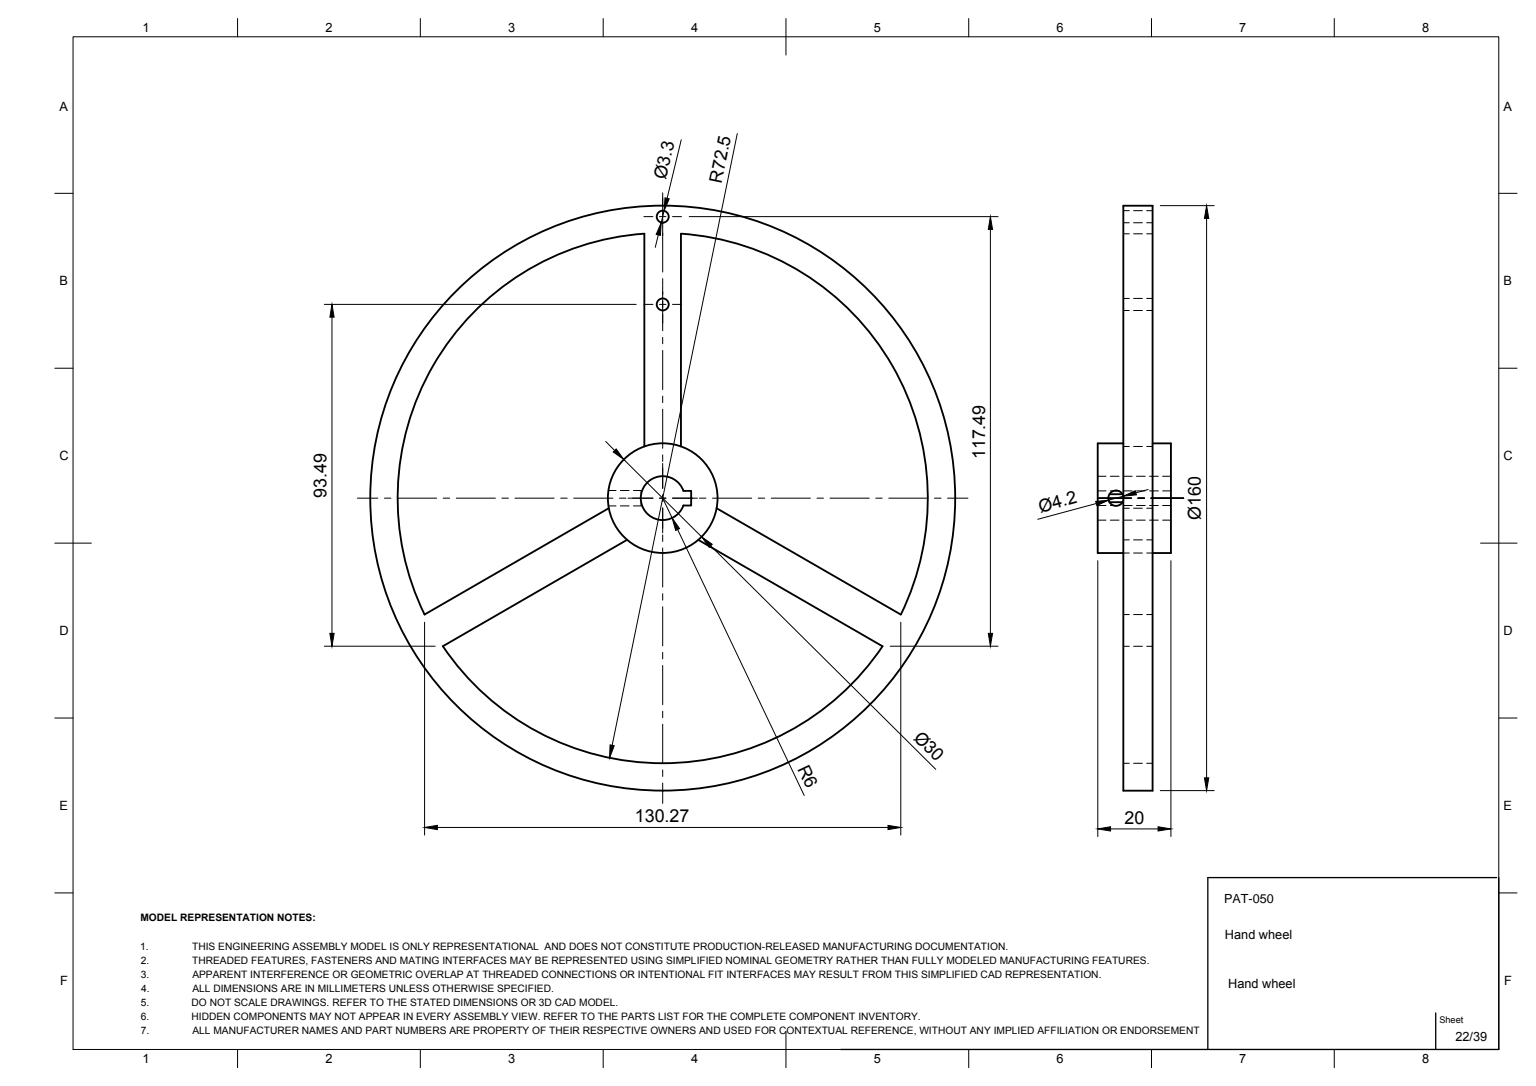
ISO-10303-21;
HEADER;
/* Generated by software containing ST-Developer
 * from STEP Tools, Inc. (www.steptools.com) 
 */

FILE_DESCRIPTION(
/* description */ ('Hand wheel with handle and shaft collar'),
/* implementation_level */ '2;1');

FILE_NAME(
/* name */ 'Hand wheel.step',
/* time_stamp */ '2026-10-28T03:23:19-07:00',
/* author */ (''),
/* organization */ (''),
/* preprocessor_version */ 'ST-DEVELOPER v20.2',
/* originating_system */ 'Autodesk Translation Framework v15.17.0.0',
/* authorisation */ '');

FILE_SCHEMA (('AUTOMOTIVE_DESIGN { 1 0 10303 214 3 1 1 }'));
ENDSEC;

DATA;
#10=MECHANICAL_DESIGN_GEOMETRIC_PRESENTATION_REPRESENTATION('',(#417),#10510);
#241=B_SPLINE_CURVE_WITH_KNOTS('',3,(#9168,#9169,#9170,#9171,#9172,#9173,
#9174,#9175,#9176,#9177),.UNSPECIFIED.,.F.,.F.,(4,2,2,2,4),(0.84783144568341,
0.878274576930948,0.958092875386314,1.03791117384168,1.06835430508922),
 .UNSPECIFIED.);
#242=B_SPLINE_CURVE_WITH_KNOTS('',3,(#9183,#9184,#9185,#9186,#9187,#9188,
#9189,#9190,#9191,#9192,#9193,#9194,#9195,#9196,#9197,#9198,#9199,#9200),
 .UNSPECIFIED.,.F.,.F.,(4,2,2,2,2,2,2,2,4),(0.,0.079216580773363,0.158433161546726,
0.23764869707457,0.316864232602414,0.396079768130259,0.475295303658103,
0.554511884431466,0.633728465204829),.UNSPECIFIED.);
#243=B_SPLINE_CURVE_WITH_KNOTS('',3,(#9201,#9202,#9203,#9204,#9205,#9206,
#9207,#9208,#9209,#9210,#9211,#9212,#9213,#9214,#9215,#9216,#9217,#9218),
 .UNSPECIFIED.,.F.,.F.,(4,2,2,2,2,2,2,2,4),(0.633728465204829,0.712945045978192,
0.792161626751555,0.871377162279399,0.950592697807243,1.02980823333509,
1.10902376886293,1.18824034963629,1.26745693040966),.UNSPECIFIED.);
#244=B_SPLINE_CURVE_WITH_KNOTS('',3,(#9221,#9222,#9223,#9224,#9225,#9226,
#9227,#9228,#9229,#9230),.UNSPECIFIED.,.F.,.F.,(4,2,2,2,4),(0.209102862092535,
0.239545993340072,0.319364291795438,0.399182590250804,0.429625721498342),
 .UNSPECIFIED.);
#346=SHAPE_REPRESENTATION_RELATIONSHIP('SRR','None',#10664,#378);
#378=ADVANCED_BREP_SHAPE_REPRESENTATION('',(#463),#10491);
#417=STYLED_ITEM('',(#10901),#463);
#463=MANIFOLD_SOLID_BREP('Body1',#5317);
#551=FACE_BOUND('',#1301,.T.);
#552=FACE_BOUND('',#1303,.T.);
#553=FACE_BOUND('',#1307,.T.);
#554=FACE_BOUND('',#1308,.T.);
#555=FACE_BOUND('',#1309,.T.);
#556=FACE_BOUND('',#1317,.T.);
#557=FACE_BOUND('',#1318,.T.);
#558=FACE_BOUND('',#1319,.T.);
#559=FACE_BOUND('',#1323,.T.);
#560=FACE_BOUND('',#1324,.T.);
#561=FACE_BOUND('',#1325,.T.);
#562=FACE_BOUND('',#1326,.T.);
#563=FACE_BOUND('',#1328,.T.);
#672=PLANE('',#6019);
#673=PLANE('',#6024);
#674=PLANE('',#6025);
#675=PLANE('',#6026);
#676=PLANE('',#6027);
#677=PLANE('',#6028);
#678=PLANE('',#6033);
#679=PLANE('',#6034);
#680=PLANE('',#6035);
#681=PLANE('',#6045);
#682=PLANE('',#6046);
#683=PLANE('',#6049);
#684=PLANE('',#6050);
#685=PLANE('',#6051);
#686=PLANE('',#6061);
#908=FACE_OUTER_BOUND('',#1292,.T.);
#909=FACE_OUTER_BOUND('',#1293,.T.);
#910=FACE_OUTER_BOUND('',#1294,.T.);
#911=FACE_OUTER_BOUND('',#1295,.T.);
#912=FACE_OUTER_BOUND('',#1296,.T.);
#913=FACE_OUTER_BOUND('',#1297,.T.);
#914=FACE_OUTER_BOUND('',#1298,.T.);
#915=FACE_OUTER_BOUND('',#1299,.T.);
#916=FACE_OUTER_BOUND('',#1300,.T.);
#917=FACE_OUTER_BOUND('',#1302,.T.);
#918=FACE_OUTER_BOUND('',#1304,.T.);
#919=FACE_OUTER_BOUND('',#1305,.T.);
#920=FACE_OUTER_BOUND('',#1306,.T.);
#921=FACE_OUTER_BOUND('',#1310,.T.);
#922=FACE_OUTER_BOUND('',#1311,.T.);
#923=FACE_OUTER_BOUND('',#1312,.T.);
#924=FACE_OUTER_BOUND('',#1313,.T.);
#925=FACE_OUTER_BOUND('',#1314,.T.);
#926=FACE_OUTER_BOUND('',#1315,.T.);
#927=FACE_OUTER_BOUND('',#1316,.T.);
#928=FACE_OUTER_BOUND('',#1320,.T.);
#929=FACE_OUTER_BOUND('',#1321,.T.);
#930=FACE_OUTER_BOUND('',#1322,.T.);
#931=FACE_OUTER_BOUND('',#1327,.T.);
#1292=EDGE_LOOP('',(#4163,#4164,#4165,#4166));
#1293=EDGE_LOOP('',(#4167,#4168,#4169,#4170));
#1294=EDGE_LOOP('',(#4171,#4172));
#1295=EDGE_LOOP('',(#4173,#4174,#4175,#4176,#4177,#4178,#4179,#4180,#4181));
#1296=EDGE_LOOP('',(#4182,#4183,#4184));
#1297=EDGE_LOOP('',(#4185,#4186,#4187,#4188));
#1298=EDGE_LOOP('',(#4189,#4190,#4191,#4192));
#1299=EDGE_LOOP('',(#4193,#4194,#4195,#4196));
#1300=EDGE_LOOP('',(#4197));
#1301=EDGE_LOOP('',(#4198,#4199,#4200,#4201));
#1302=EDGE_LOOP('',(#4202,#4203,#4204,#4205));
#1303=EDGE_LOOP('',(#4206,#4207,#4208,#4209));
#1304=EDGE_LOOP('',(#4210,#4211,#4212,#4213));
#1305=EDGE_LOOP('',(#4214,#4215,#4216,#4217));
#1306=EDGE_LOOP('',(#4218));
#1307=EDGE_LOOP('',(#4219));
#1308=EDGE_LOOP('',(#4220));
#1309=EDGE_LOOP('',(#4221,#4222,#4223,#4224,#4225,#4226,#4227,#4228,#4229,
#4230,#4231,#4232));
#1310=EDGE_LOOP('',(#4233,#4234,#4235,#4236));
#1311=EDGE_LOOP('',(#4237,#4238,#4239,#4240));
#1312=EDGE_LOOP('',(#4241,#4242,#4243,#4244));
#1313=EDGE_LOOP('',(#4245,#4246,#4247,#4248));
#1314=EDGE_LOOP('',(#4249,#4250,#4251,#4252));
#1315=EDGE_LOOP('',(#4253,#4254,#4255,#4256));
#1316=EDGE_LOOP('',(#4257));
#1317=EDGE_LOOP('',(#4258));
#1318=EDGE_LOOP('',(#4259));
#1319=EDGE_LOOP('',(#4260,#4261,#4262,#4263,#4264,#4265,#4266,#4267,#4268,
#4269,#4270,#4271));
#1320=EDGE_LOOP('',(#4272,#4273,#4274,#4275));
#1321=EDGE_LOOP('',(#4276,#4277,#4278,#4279));
#1322=EDGE_LOOP('',(#4280,#4281,#4282,#4283));
#1323=EDGE_LOOP('',(#4284,#4285));
#1324=EDGE_LOOP('',(#4286,#4287,#4288,#4289));
#1325=EDGE_LOOP('',(#4290,#4291,#4292,#4293));
#1326=EDGE_LOOP('',(#4294,#4295,#4296,#4297));
#1327=EDGE_LOOP('',(#4298));
#1328=EDGE_LOOP('',(#4299,#4300,#4301,#4302));
#1656=LINE('',#9153,#1966);
#1657=LINE('',#9159,#1967);
#1658=LINE('',#9164,#1968);
#1659=LINE('',#9181,#1969);
#1660=LINE('',#9232,#1970);
#1661=LINE('',#9236,#1971);
#1662=LINE('',#9238,#1972);
#1663=LINE('',#9240,#1973);
#1664=LINE('',#9241,#1974);
#1665=LINE('',#9244,#1975);
#1666=LINE('',#9246,#1976);
#1667=LINE('',#9247,#1977);
#1668=LINE('',#9250,#1978);
#1669=LINE('',#9252,#1979);
#1670=LINE('',#9253,#1980);
#1671=LINE('',#9263,#1981);
#1672=LINE('',#9265,#1982);
#1673=LINE('',#9267,#1983);
#1674=LINE('',#9268,#1984);
#1675=LINE('',#9272,#1985);
#1676=LINE('',#9274,#1986);
#1677=LINE('',#9276,#1987);
#1678=LINE('',#9277,#1988);
#1679=LINE('',#9284,#1989);
#1680=LINE('',#9288,#1990);
#1681=LINE('',#9292,#1991);
#1682=LINE('',#9296,#1992);
#1683=LINE('',#9302,#1993);
#1684=LINE('',#9305,#1994);
#1685=LINE('',#9306,#1995);
#1686=LINE('',#9309,#1996);
#1687=LINE('',#9311,#1997);
#1688=LINE('',#9312,#1998);
#1689=LINE('',#9316,#1999);
#1690=LINE('',#9319,#2000);
#1691=LINE('',#9320,#2001);
#1692=LINE('',#9323,#2002);
#1693=LINE('',#9325,#2003);
#1694=LINE('',#9326,#2004);
#1695=LINE('',#9336,#2005);
#1696=LINE('',#9339,#2006);
#1966=VECTOR('',#7198,0.165);
#1967=VECTOR('',#7205,0.165);
#1968=VECTOR('',#7210,1.);
#1969=VECTOR('',#7217,0.21);
#1970=VECTOR('',#7222,1.);
#1971=VECTOR('',#7225,1.);
#1972=VECTOR('',#7226,1.);
#1973=VECTOR('',#7227,1.);
#1974=VECTOR('',#7228,1.);
#1975=VECTOR('',#7231,1.);
#1976=VECTOR('',#7232,1.);
#1977=VECTOR('',#7233,1.);
#1978=VECTOR('',#7236,1.);
#1979=VECTOR('',#7237,1.);
#1980=VECTOR('',#7238,1.);
#1981=VECTOR('',#7251,1.);
#1982=VECTOR('',#7252,1.);
#1983=VECTOR('',#7253,1.);
#1984=VECTOR('',#7254,1.);
#1985=VECTOR('',#7257,1.);
#1986=VECTOR('',#7258,1.);
#1987=VECTOR('',#7259,1.);
#1988=VECTOR('',#7260,1.);
#1989=VECTOR('',#7267,1.);
#1990=VECTOR('',#7270,1.);
#1991=VECTOR('',#7273,1.);
#1992=VECTOR('',#7276,1.);
#1993=VECTOR('',#7285,1.);
#1994=VECTOR('',#7288,1.);
#1995=VECTOR('',#7289,1.);
#1996=VECTOR('',#7292,1.);
#1997=VECTOR('',#7293,1.);
#1998=VECTOR('',#7294,1.);
#1999=VECTOR('',#7299,1.);
#2000=VECTOR('',#7302,1.);
#2001=VECTOR('',#7303,1.);
#2002=VECTOR('',#7306,1.);
#2003=VECTOR('',#7307,1.);
#2004=VECTOR('',#7308,1.);
#2005=VECTOR('',#7325,8.);
#2006=VECTOR('',#7328,1.5);
#2279=CIRCLE('',#6014,0.165);
#2280=CIRCLE('',#6015,0.165);
#2281=CIRCLE('',#6017,0.165);
#2282=CIRCLE('',#6018,0.165);
#2283=CIRCLE('',#6020,0.21);
#2284=CIRCLE('',#6022,0.21);
#2285=CIRCLE('',#6023,0.21);
#2286=CIRCLE('',#6029,1.5);
#2287=CIRCLE('',#6030,0.6);
#2288=CIRCLE('',#6032,0.6);
#2289=CIRCLE('',#6036,8.);
#2290=CIRCLE('',#6037,7.25);
#2291=CIRCLE('',#6038,1.5);
#2292=CIRCLE('',#6039,7.25);
#2293=CIRCLE('',#6040,1.5);
#2294=CIRCLE('',#6041,7.25);
#2295=CIRCLE('',#6042,1.5);
#2296=CIRCLE('',#6044,7.25);
#2297=CIRCLE('',#6048,7.25);
#2298=CIRCLE('',#6052,8.);
#2299=CIRCLE('',#6053,7.25);
#2300=CIRCLE('',#6054,1.5);
#2301=CIRCLE('',#6055,1.5);
#2302=CIRCLE('',#6056,1.5);
#2303=CIRCLE('',#6060,1.5);
#2653=VERTEX_POINT('',#9150);
#2654=VERTEX_POINT('',#9152);
#2655=VERTEX_POINT('',#9156);
#2656=VERTEX_POINT('',#9158);
#2657=VERTEX_POINT('',#9162);
#2658=VERTEX_POINT('',#9163);
#2659=VERTEX_POINT('',#9167);
#2660=VERTEX_POINT('',#9178);
#2661=VERTEX_POINT('',#9180);
#2662=VERTEX_POINT('',#9182);
#2663=VERTEX_POINT('',#9219);
#2664=VERTEX_POINT('',#9234);
#2665=VERTEX_POINT('',#9235);
#2666=VERTEX_POINT('',#9237);
#2667=VERTEX_POINT('',#9239);
#2668=VERTEX_POINT('',#9243);
#2669=VERTEX_POINT('',#9245);
#2670=VERTEX_POINT('',#9249);
#2671=VERTEX_POINT('',#9251);
#2672=VERTEX_POINT('',#9255);
#2673=VERTEX_POINT('',#9261);
#2674=VERTEX_POINT('',#9262);
#2675=VERTEX_POINT('',#9264);
#2676=VERTEX_POINT('',#9266);
#2677=VERTEX_POINT('',#9270);
#2678=VERTEX_POINT('',#9271);
#2679=VERTEX_POINT('',#9273);
#2680=VERTEX_POINT('',#9275);
#2681=VERTEX_POINT('',#9279);
#2682=VERTEX_POINT('',#9281);
#2683=VERTEX_POINT('',#9283);
#2684=VERTEX_POINT('',#9285);
#2685=VERTEX_POINT('',#9287);
#2686=VERTEX_POINT('',#9289);
#2687=VERTEX_POINT('',#9291);
#2688=VERTEX_POINT('',#9293);
#2689=VERTEX_POINT('',#9295);
#2690=VERTEX_POINT('',#9300);
#2691=VERTEX_POINT('',#9304);
#2692=VERTEX_POINT('',#9308);
#2693=VERTEX_POINT('',#9310);
#2694=VERTEX_POINT('',#9314);
#2695=VERTEX_POINT('',#9318);
#2696=VERTEX_POINT('',#9322);
#2697=VERTEX_POINT('',#9324);
#2698=VERTEX_POINT('',#9328);
#2699=VERTEX_POINT('',#9338);
#3199=EDGE_CURVE('',#2653,#2653,#2279,.T.);
#3200=EDGE_CURVE('',#2653,#2654,#1656,.T.);
#3201=EDGE_CURVE('',#2654,#2654,#2280,.T.);
#3202=EDGE_CURVE('',#2655,#2655,#2281,.T.);
#3203=EDGE_CURVE('',#2655,#2656,#1657,.T.);
#3204=EDGE_CURVE('',#2656,#2656,#2282,.T.);
#3205=EDGE_CURVE('',#2657,#2658,#1658,.T.);
#3206=EDGE_CURVE('',#2657,#2658,#2283,.T.);
#3207=EDGE_CURVE('',#2659,#2657,#241,.T.);
#3208=EDGE_CURVE('',#2660,#2659,#2284,.T.);
#3209=EDGE_CURVE('',#2660,#2661,#1659,.T.);
#3210=EDGE_CURVE('',#2662,#2661,#242,.T.);
#3211=EDGE_CURVE('',#2661,#2662,#243,.T.);
#3212=EDGE_CURVE('',#2663,#2660,#2285,.T.);
#3213=EDGE_CURVE('',#2658,#2663,#244,.T.);
#3214=EDGE_CURVE('',#2663,#2659,#1660,.T.);
#3215=EDGE_CURVE('',#2664,#2665,#1661,.T.);
#3216=EDGE_CURVE('',#2664,#2666,#1662,.T.);
#3217=EDGE_CURVE('',#2667,#2666,#1663,.T.);
#3218=EDGE_CURVE('',#2665,#2667,#1664,.T.);
#3219=EDGE_CURVE('',#2668,#2664,#1665,.T.);
#3220=EDGE_CURVE('',#2668,#2669,#1666,.T.);
#3221=EDGE_CURVE('',#2666,#2669,#1667,.T.);
#3222=EDGE_CURVE('',#2670,#2668,#1668,.T.);
#3223=EDGE_CURVE('',#2671,#2670,#1669,.T.);
#3224=EDGE_CURVE('',#2669,#2671,#1670,.T.);
#3225=EDGE_CURVE('',#2672,#2672,#2286,.T.);
#3226=EDGE_CURVE('',#2671,#2667,#2287,.T.);
#3227=EDGE_CURVE('',#2670,#2665,#2288,.T.);
#3228=EDGE_CURVE('',#2673,#2674,#1671,.T.);
#3229=EDGE_CURVE('',#2675,#2673,#1672,.T.);
#3230=EDGE_CURVE('',#2676,#2675,#1673,.T.);
#3231=EDGE_CURVE('',#2674,#2676,#1674,.T.);
#3232=EDGE_CURVE('',#2677,#2678,#1675,.T.);
#3233=EDGE_CURVE('',#2679,#2677,#1676,.T.);
#3234=EDGE_CURVE('',#2680,#2679,#1677,.T.);
#3235=EDGE_CURVE('',#2678,#2680,#1678,.T.);
#3236=EDGE_CURVE('',#2681,#2681,#2289,.T.);
#3237=EDGE_CURVE('',#2682,#2677,#2290,.T.);
#3238=EDGE_CURVE('',#2682,#2683,#1679,.T.);
#3239=EDGE_CURVE('',#2684,#2683,#2291,.T.);
#3240=EDGE_CURVE('',#2684,#2685,#1680,.T.);
#3241=EDGE_CURVE('',#2686,#2685,#2292,.T.);
#3242=EDGE_CURVE('',#2686,#2687,#1681,.T.);
#3243=EDGE_CURVE('',#2688,#2687,#2293,.T.);
#3244=EDGE_CURVE('',#2688,#2689,#1682,.T.);
#3245=EDGE_CURVE('',#2674,#2689,#2294,.T.);
#3246=EDGE_CURVE('',#2679,#2676,#2295,.T.);
#3247=EDGE_CURVE('',#2690,#2678,#2296,.T.);
#3248=EDGE_CURVE('',#2690,#2682,#1683,.T.);
#3249=EDGE_CURVE('',#2691,#2690,#1684,.T.);
#3250=EDGE_CURVE('',#2683,#2691,#1685,.T.);
#3251=EDGE_CURVE('',#2685,#2692,#1686,.T.);
#3252=EDGE_CURVE('',#2693,#2684,#1687,.T.);
#3253=EDGE_CURVE('',#2692,#2693,#1688,.T.);
#3254=EDGE_CURVE('',#2694,#2692,#2297,.T.);
#3255=EDGE_CURVE('',#2694,#2686,#1689,.T.);
#3256=EDGE_CURVE('',#2687,#2695,#1690,.T.);
#3257=EDGE_CURVE('',#2695,#2694,#1691,.T.);
#3258=EDGE_CURVE('',#2696,#2688,#1692,.T.);
#3259=EDGE_CURVE('',#2697,#2696,#1693,.T.);
#3260=EDGE_CURVE('',#2689,#2697,#1694,.T.);
#3261=EDGE_CURVE('',#2698,#2698,#2298,.T.);
#3262=EDGE_CURVE('',#2673,#2697,#2299,.T.);
#3263=EDGE_CURVE('',#2695,#2696,#2300,.T.);
#3264=EDGE_CURVE('',#2691,#2693,#2301,.T.);
#3265=EDGE_CURVE('',#2675,#2680,#2302,.T.);
#3266=EDGE_CURVE('',#2698,#2681,#1695,.T.);
#3267=EDGE_CURVE('',#2672,#2699,#1696,.T.);
#3268=EDGE_CURVE('',#2699,#2699,#2303,.T.);
#4163=ORIENTED_EDGE('',*,*,#3199,.F.);
#4164=ORIENTED_EDGE('',*,*,#3200,.T.);
#4165=ORIENTED_EDGE('',*,*,#3201,.F.);
#4166=ORIENTED_EDGE('',*,*,#3200,.F.);
#4167=ORIENTED_EDGE('',*,*,#3202,.F.);
#4168=ORIENTED_EDGE('',*,*,#3203,.T.);
#4169=ORIENTED_EDGE('',*,*,#3204,.F.);
#4170=ORIENTED_EDGE('',*,*,#3203,.F.);
#4171=ORIENTED_EDGE('',*,*,#3205,.F.);
#4172=ORIENTED_EDGE('',*,*,#3206,.T.);
#4173=ORIENTED_EDGE('',*,*,#3207,.F.);
#4174=ORIENTED_EDGE('',*,*,#3208,.F.);
#4175=ORIENTED_EDGE('',*,*,#3209,.T.);
#4176=ORIENTED_EDGE('',*,*,#3210,.F.);
#4177=ORIENTED_EDGE('',*,*,#3211,.F.);
#4178=ORIENTED_EDGE('',*,*,#3209,.F.);
#4179=ORIENTED_EDGE('',*,*,#3212,.F.);
#4180=ORIENTED_EDGE('',*,*,#3213,.F.);
#4181=ORIENTED_EDGE('',*,*,#3206,.F.);
#4182=ORIENTED_EDGE('',*,*,#3214,.F.);
#4183=ORIENTED_EDGE('',*,*,#3212,.T.);
#4184=ORIENTED_EDGE('',*,*,#3208,.T.);
#4185=ORIENTED_EDGE('',*,*,#3215,.F.);
#4186=ORIENTED_EDGE('',*,*,#3216,.T.);
#4187=ORIENTED_EDGE('',*,*,#3217,.F.);
#4188=ORIENTED_EDGE('',*,*,#3218,.F.);
#4189=ORIENTED_EDGE('',*,*,#3219,.F.);
#4190=ORIENTED_EDGE('',*,*,#3220,.T.);
#4191=ORIENTED_EDGE('',*,*,#3221,.F.);
#4192=ORIENTED_EDGE('',*,*,#3216,.F.);
#4193=ORIENTED_EDGE('',*,*,#3222,.F.);
#4194=ORIENTED_EDGE('',*,*,#3223,.F.);
#4195=ORIENTED_EDGE('',*,*,#3224,.F.);
#4196=ORIENTED_EDGE('',*,*,#3220,.F.);
#4197=ORIENTED_EDGE('',*,*,#3225,.T.);
#4198=ORIENTED_EDGE('',*,*,#3217,.T.);
#4199=ORIENTED_EDGE('',*,*,#3221,.T.);
#4200=ORIENTED_EDGE('',*,*,#3224,.T.);
#4201=ORIENTED_EDGE('',*,*,#3226,.T.);
#4202=ORIENTED_EDGE('',*,*,#3218,.T.);
#4203=ORIENTED_EDGE('',*,*,#3226,.F.);
#4204=ORIENTED_EDGE('',*,*,#3223,.T.);
#4205=ORIENTED_EDGE('',*,*,#3227,.T.);
#4206=ORIENTED_EDGE('',*,*,#3213,.T.);
#4207=ORIENTED_EDGE('',*,*,#3214,.T.);
#4208=ORIENTED_EDGE('',*,*,#3207,.T.);
#4209=ORIENTED_EDGE('',*,*,#3205,.T.);
#4210=ORIENTED_EDGE('',*,*,#3228,.F.);
#4211=ORIENTED_EDGE('',*,*,#3229,.F.);
#4212=ORIENTED_EDGE('',*,*,#3230,.F.);
#4213=ORIENTED_EDGE('',*,*,#3231,.F.);
#4214=ORIENTED_EDGE('',*,*,#3232,.F.);
#4215=ORIENTED_EDGE('',*,*,#3233,.F.);
#4216=ORIENTED_EDGE('',*,*,#3234,.F.);
#4217=ORIENTED_EDGE('',*,*,#3235,.F.);
#4218=ORIENTED_EDGE('',*,*,#3236,.F.);
#4219=ORIENTED_EDGE('',*,*,#3199,.T.);
#4220=ORIENTED_EDGE('',*,*,#3202,.T.);
#4221=ORIENTED_EDGE('',*,*,#3237,.F.);
#4222=ORIENTED_EDGE('',*,*,#3238,.T.);
#4223=ORIENTED_EDGE('',*,*,#3239,.F.);
#4224=ORIENTED_EDGE('',*,*,#3240,.T.);
#4225=ORIENTED_EDGE('',*,*,#3241,.F.);
#4226=ORIENTED_EDGE('',*,*,#3242,.T.);
#4227=ORIENTED_EDGE('',*,*,#3243,.F.);
#4228=ORIENTED_EDGE('',*,*,#3244,.T.);
#4229=ORIENTED_EDGE('',*,*,#3245,.F.);
#4230=ORIENTED_EDGE('',*,*,#3231,.T.);
#4231=ORIENTED_EDGE('',*,*,#3246,.F.);
#4232=ORIENTED_EDGE('',*,*,#3233,.T.);
#4233=ORIENTED_EDGE('',*,*,#3232,.T.);
#4234=ORIENTED_EDGE('',*,*,#3247,.F.);
#4235=ORIENTED_EDGE('',*,*,#3248,.T.);
#4236=ORIENTED_EDGE('',*,*,#3237,.T.);
#4237=ORIENTED_EDGE('',*,*,#3248,.F.);
#4238=ORIENTED_EDGE('',*,*,#3249,.F.);
#4239=ORIENTED_EDGE('',*,*,#3250,.F.);
#4240=ORIENTED_EDGE('',*,*,#3238,.F.);
#4241=ORIENTED_EDGE('',*,*,#3251,.F.);
#4242=ORIENTED_EDGE('',*,*,#3240,.F.);
#4243=ORIENTED_EDGE('',*,*,#3252,.F.);
#4244=ORIENTED_EDGE('',*,*,#3253,.F.);
#4245=ORIENTED_EDGE('',*,*,#3251,.T.);
#4246=ORIENTED_EDGE('',*,*,#3254,.F.);
#4247=ORIENTED_EDGE('',*,*,#3255,.T.);
#4248=ORIENTED_EDGE('',*,*,#3241,.T.);
#4249=ORIENTED_EDGE('',*,*,#3256,.F.);
#4250=ORIENTED_EDGE('',*,*,#3242,.F.);
#4251=ORIENTED_EDGE('',*,*,#3255,.F.);
#4252=ORIENTED_EDGE('',*,*,#3257,.F.);
#4253=ORIENTED_EDGE('',*,*,#3258,.F.);
#4254=ORIENTED_EDGE('',*,*,#3259,.F.);
#4255=ORIENTED_EDGE('',*,*,#3260,.F.);
#4256=ORIENTED_EDGE('',*,*,#3244,.F.);
#4257=ORIENTED_EDGE('',*,*,#3261,.T.);
#4258=ORIENTED_EDGE('',*,*,#3201,.T.);
#4259=ORIENTED_EDGE('',*,*,#3204,.T.);
#4260=ORIENTED_EDGE('',*,*,#3262,.T.);
#4261=ORIENTED_EDGE('',*,*,#3259,.T.);
#4262=ORIENTED_EDGE('',*,*,#3263,.F.);
#4263=ORIENTED_EDGE('',*,*,#3257,.T.);
#4264=ORIENTED_EDGE('',*,*,#3254,.T.);
#4265=ORIENTED_EDGE('',*,*,#3253,.T.);
#4266=ORIENTED_EDGE('',*,*,#3264,.F.);
#4267=ORIENTED_EDGE('',*,*,#3249,.T.);
#4268=ORIENTED_EDGE('',*,*,#3247,.T.);
#4269=ORIENTED_EDGE('',*,*,#3235,.T.);
#4270=ORIENTED_EDGE('',*,*,#3265,.F.);
#4271=ORIENTED_EDGE('',*,*,#3229,.T.);
#4272=ORIENTED_EDGE('',*,*,#3228,.T.);
#4273=ORIENTED_EDGE('',*,*,#3245,.T.);
#4274=ORIENTED_EDGE('',*,*,#3260,.T.);
#4275=ORIENTED_EDGE('',*,*,#3262,.F.);
#4276=ORIENTED_EDGE('',*,*,#3261,.F.);
#4277=ORIENTED_EDGE('',*,*,#3266,.T.);
#4278=ORIENTED_EDGE('',*,*,#3236,.T.);
#4279=ORIENTED_EDGE('',*,*,#3266,.F.);
#4280=ORIENTED_EDGE('',*,*,#3225,.F.);
#4281=ORIENTED_EDGE('',*,*,#3267,.T.);
#4282=ORIENTED_EDGE('',*,*,#3268,.T.);
#4283=ORIENTED_EDGE('',*,*,#3267,.F.);
#4284=ORIENTED_EDGE('',*,*,#3210,.T.);
#4285=ORIENTED_EDGE('',*,*,#3211,.T.);
#4286=ORIENTED_EDGE('',*,*,#3230,.T.);
#4287=ORIENTED_EDGE('',*,*,#3265,.T.);
#4288=ORIENTED_EDGE('',*,*,#3234,.T.);
#4289=ORIENTED_EDGE('',*,*,#3246,.T.);
#4290=ORIENTED_EDGE('',*,*,#3250,.T.);
#4291=ORIENTED_EDGE('',*,*,#3264,.T.);
#4292=ORIENTED_EDGE('',*,*,#3252,.T.);
#4293=ORIENTED_EDGE('',*,*,#3239,.T.);
#4294=ORIENTED_EDGE('',*,*,#3256,.T.);
#4295=ORIENTED_EDGE('',*,*,#3263,.T.);
#4296=ORIENTED_EDGE('',*,*,#3258,.T.);
#4297=ORIENTED_EDGE('',*,*,#3243,.T.);
#4298=ORIENTED_EDGE('',*,*,#3268,.F.);
#4299=ORIENTED_EDGE('',*,*,#3215,.T.);
#4300=ORIENTED_EDGE('',*,*,#3227,.F.);
#4301=ORIENTED_EDGE('',*,*,#3222,.T.);
#4302=ORIENTED_EDGE('',*,*,#3219,.T.);
#4927=CYLINDRICAL_SURFACE('',#6013,0.165);
#4928=CYLINDRICAL_SURFACE('',#6016,0.165);
#4929=CYLINDRICAL_SURFACE('',#6021,0.21);
#4930=CYLINDRICAL_SURFACE('',#6031,0.6);
#4931=CYLINDRICAL_SURFACE('',#6043,7.25);
#4932=CYLINDRICAL_SURFACE('',#6047,7.25);
#4933=CYLINDRICAL_SURFACE('',#6057,7.25);
#4934=CYLINDRICAL_SURFACE('',#6058,8.);
#4935=CYLINDRICAL_SURFACE('',#6059,1.5);
#5120=ADVANCED_FACE('',(#908),#4927,.F.);
#5121=ADVANCED_FACE('',(#909),#4928,.F.);
#5122=ADVANCED_FACE('',(#910),#672,.T.);
#5123=ADVANCED_FACE('',(#911),#4929,.F.);
#5124=ADVANCED_FACE('',(#912),#673,.T.);
#5125=ADVANCED_FACE('',(#913),#674,.F.);
#5126=ADVANCED_FACE('',(#914),#675,.F.);
#5127=ADVANCED_FACE('',(#915),#676,.F.);
#5128=ADVANCED_FACE('',(#916,#551),#677,.T.);
#5129=ADVANCED_FACE('',(#917,#552),#4930,.F.);
#5130=ADVANCED_FACE('',(#918),#678,.T.);
#5131=ADVANCED_FACE('',(#919),#679,.T.);
#5132=ADVANCED_FACE('',(#920,#553,#554,#555),#680,.F.);
#5133=ADVANCED_FACE('',(#921),#4931,.F.);
#5134=ADVANCED_FACE('',(#922),#681,.T.);
#5135=ADVANCED_FACE('',(#923),#682,.T.);
#5136=ADVANCED_FACE('',(#924),#4932,.F.);
#5137=ADVANCED_FACE('',(#925),#683,.T.);
#5138=ADVANCED_FACE('',(#926),#684,.T.);
#5139=ADVANCED_FACE('',(#927,#556,#557,#558),#685,.T.);
#5140=ADVANCED_FACE('',(#928),#4933,.F.);
#5141=ADVANCED_FACE('',(#929),#4934,.T.);
#5142=ADVANCED_FACE('',(#930,#559,#560,#561,#562),#4935,.T.);
#5143=ADVANCED_FACE('',(#931,#563),#686,.F.);
#5317=CLOSED_SHELL('',(#5120,#5121,#5122,#5123,#5124,#5125,#5126,#5127,
#5128,#5129,#5130,#5131,#5132,#5133,#5134,#5135,#5136,#5137,#5138,#5139,
#5140,#5141,#5142,#5143));
#6012=AXIS2_PLACEMENT_3D('',#9148,#7192,#7193);
#6013=AXIS2_PLACEMENT_3D('',#9149,#7194,#7195);
#6014=AXIS2_PLACEMENT_3D('',#9151,#7196,#7197);
#6015=AXIS2_PLACEMENT_3D('',#9154,#7199,#7200);
#6016=AXIS2_PLACEMENT_3D('',#9155,#7201,#7202);
#6017=AXIS2_PLACEMENT_3D('',#9157,#7203,#7204);
#6018=AXIS2_PLACEMENT_3D('',#9160,#7206,#7207);
#6019=AXIS2_PLACEMENT_3D('',#9161,#7208,#7209);
#6020=AXIS2_PLACEMENT_3D('',#9165,#7211,#7212);
#6021=AXIS2_PLACEMENT_3D('',#9166,#7213,#7214);
#6022=AXIS2_PLACEMENT_3D('',#9179,#7215,#7216);
#6023=AXIS2_PLACEMENT_3D('',#9220,#7218,#7219);
#6024=AXIS2_PLACEMENT_3D('',#9231,#7220,#7221);
#6025=AXIS2_PLACEMENT_3D('',#9233,#7223,#7224);
#6026=AXIS2_PLACEMENT_3D('',#9242,#7229,#7230);
#6027=AXIS2_PLACEMENT_3D('',#9248,#7234,#7235);
#6028=AXIS2_PLACEMENT_3D('',#9254,#7239,#7240);
#6029=AXIS2_PLACEMENT_3D('',#9256,#7241,#7242);
#6030=AXIS2_PLACEMENT_3D('',#9257,#7243,#7244);
#6031=AXIS2_PLACEMENT_3D('',#9258,#7245,#7246);
#6032=AXIS2_PLACEMENT_3D('',#9259,#7247,#7248);
#6033=AXIS2_PLACEMENT_3D('',#9260,#7249,#7250);
#6034=AXIS2_PLACEMENT_3D('',#9269,#7255,#7256);
#6035=AXIS2_PLACEMENT_3D('',#9278,#7261,#7262);
#6036=AXIS2_PLACEMENT_3D('',#9280,#7263,#7264);
#6037=AXIS2_PLACEMENT_3D('',#9282,#7265,#7266);
#6038=AXIS2_PLACEMENT_3D('',#9286,#7268,#7269);
#6039=AXIS2_PLACEMENT_3D('',#9290,#7271,#7272);
#6040=AXIS2_PLACEMENT_3D('',#9294,#7274,#7275);
#6041=AXIS2_PLACEMENT_3D('',#9297,#7277,#7278);
#6042=AXIS2_PLACEMENT_3D('',#9298,#7279,#7280);
#6043=AXIS2_PLACEMENT_3D('',#9299,#7281,#7282);
#6044=AXIS2_PLACEMENT_3D('',#9301,#7283,#7284);
#6045=AXIS2_PLACEMENT_3D('',#9303,#7286,#7287);
#6046=AXIS2_PLACEMENT_3D('',#9307,#7290,#7291);
#6047=AXIS2_PLACEMENT_3D('',#9313,#7295,#7296);
#6048=AXIS2_PLACEMENT_3D('',#9315,#7297,#7298);
#6049=AXIS2_PLACEMENT_3D('',#9317,#7300,#7301);
#6050=AXIS2_PLACEMENT_3D('',#9321,#7304,#7305);
#6051=AXIS2_PLACEMENT_3D('',#9327,#7309,#7310);
#6052=AXIS2_PLACEMENT_3D('',#9329,#7311,#7312);
#6053=AXIS2_PLACEMENT_3D('',#9330,#7313,#7314);
#6054=AXIS2_PLACEMENT_3D('',#9331,#7315,#7316);
#6055=AXIS2_PLACEMENT_3D('',#9332,#7317,#7318);
#6056=AXIS2_PLACEMENT_3D('',#9333,#7319,#7320);
#6057=AXIS2_PLACEMENT_3D('',#9334,#7321,#7322);
#6058=AXIS2_PLACEMENT_3D('',#9335,#7323,#7324);
#6059=AXIS2_PLACEMENT_3D('',#9337,#7326,#7327);
#6060=AXIS2_PLACEMENT_3D('',#9340,#7329,#7330);
#6061=AXIS2_PLACEMENT_3D('',#9341,#7331,#7332);
#7192=DIRECTION('axis',(0.,0.,1.));
#7193=DIRECTION('refdir',(1.,0.,0.));
#7194=DIRECTION('center_axis',(0.,1.,0.));
#7195=DIRECTION('ref_axis',(1.,0.,0.));
#7196=DIRECTION('center_axis',(0.,1.,0.));
#7197=DIRECTION('ref_axis',(1.,0.,0.));
#7198=DIRECTION('',(0.,1.,0.));
#7199=DIRECTION('center_axis',(0.,-1.,0.));
#7200=DIRECTION('ref_axis',(1.,0.,0.));
#7201=DIRECTION('center_axis',(0.,1.,0.));
#7202=DIRECTION('ref_axis',(1.,0.,0.));
#7203=DIRECTION('center_axis',(0.,1.,0.));
#7204=DIRECTION('ref_axis',(1.,0.,0.));
#7205=DIRECTION('',(0.,1.,0.));
#7206=DIRECTION('center_axis',(0.,-1.,0.));
#7207=DIRECTION('ref_axis',(1.,0.,0.));
#7208=DIRECTION('center_axis',(0.,0.,1.));
#7209=DIRECTION('ref_axis',(1.,0.,0.));
#7210=DIRECTION('',(0.,1.,0.));
#7211=DIRECTION('center_axis',(0.,0.,1.));
#7212=DIRECTION('ref_axis',(1.,0.,0.));
#7213=DIRECTION('center_axis',(0.,0.,1.));
#7214=DIRECTION('ref_axis',(1.,0.,0.));
#7215=DIRECTION('center_axis',(0.,0.,1.));
#7216=DIRECTION('ref_axis',(1.,0.,0.));
#7217=DIRECTION('',(0.,0.,1.));
#7218=DIRECTION('center_axis',(0.,0.,1.));
#7219=DIRECTION('ref_axis',(1.,0.,0.));
#7220=DIRECTION('center_axis',(0.,0.,1.));
#7221=DIRECTION('ref_axis',(1.,0.,0.));
#7222=DIRECTION('',(0.,-1.,0.));
#7223=DIRECTION('center_axis',(-1.,0.,0.));
#7224=DIRECTION('ref_axis',(0.,0.,1.));
#7225=DIRECTION('',(0.,0.,1.));
#7226=DIRECTION('',(0.,1.,0.));
#7227=DIRECTION('',(0.,0.,-1.));
#7228=DIRECTION('',(0.,1.,0.));
#7229=DIRECTION('center_axis',(0.,0.,-1.));
#7230=DIRECTION('ref_axis',(-1.,0.,0.));
#7231=DIRECTION('',(-1.,0.,0.));
#7232=DIRECTION('',(0.,1.,0.));
#7233=DIRECTION('',(1.,0.,0.));
#7234=DIRECTION('center_axis',(1.,0.,0.));
#7235=DIRECTION('ref_axis',(0.,0.,-1.));
#7236=DIRECTION('',(0.,0.,-1.));
#7237=DIRECTION('',(0.,-1.,0.));
#7238=DIRECTION('',(0.,0.,1.));
#7239=DIRECTION('center_axis',(0.,1.,0.));
#7240=DIRECTION('ref_axis',(1.,0.,0.));
#7241=DIRECTION('center_axis',(0.,1.,0.));
#7242=DIRECTION('ref_axis',(1.,0.,0.));
#7243=DIRECTION('center_axis',(0.,-1.,0.));
#7244=DIRECTION('ref_axis',(1.,0.,0.));
#7245=DIRECTION('center_axis',(0.,1.,0.));
#7246=DIRECTION('ref_axis',(-1.83697019872103E-16,0.,1.));
#7247=DIRECTION('center_axis',(0.,-1.,0.));
#7248=DIRECTION('ref_axis',(1.,0.,0.));
#7249=DIRECTION('center_axis',(0.866025403784438,0.,-0.5));
#7250=DIRECTION('ref_axis',(-0.5,0.,-0.866025403784438));
#7251=DIRECTION('',(0.,-1.,0.));
#7252=DIRECTION('',(-0.5,0.,-0.866025403784438));
#7253=DIRECTION('',(0.,1.,0.));
#7254=DIRECTION('',(0.5,0.,0.866025403784438));
#7255=DIRECTION('center_axis',(-0.866025403784438,0.,0.5));
#7256=DIRECTION('ref_axis',(0.5,0.,0.866025403784438));
#7257=DIRECTION('',(0.,1.,0.));
#7258=DIRECTION('',(-0.5,0.,-0.866025403784438));
#7259=DIRECTION('',(0.,-1.,0.));
#7260=DIRECTION('',(0.5,0.,0.866025403784438));
#7261=DIRECTION('center_axis',(0.,1.,0.));
#7262=DIRECTION('ref_axis',(1.,0.,0.));
#7263=DIRECTION('center_axis',(0.,1.,0.));
#7264=DIRECTION('ref_axis',(1.,0.,0.));
#7265=DIRECTION('center_axis',(0.,-1.,0.));
#7266=DIRECTION('ref_axis',(1.,0.,0.));
#7267=DIRECTION('',(0.5,0.,-0.866025403784439));
#7268=DIRECTION('center_axis',(0.,-1.,0.));
#7269=DIRECTION('ref_axis',(1.,0.,0.));
#7270=DIRECTION('',(-0.5,0.,0.866025403784439));
#7271=DIRECTION('center_axis',(0.,-1.,0.));
#7272=DIRECTION('ref_axis',(1.,0.,0.));
#7273=DIRECTION('',(-1.,0.,0.));
#7274=DIRECTION('center_axis',(0.,-1.,0.));
#7275=DIRECTION('ref_axis',(1.,0.,0.));
#7276=DIRECTION('',(1.,0.,0.));
#7277=DIRECTION('center_axis',(0.,-1.,0.));
#7278=DIRECTION('ref_axis',(1.,0.,0.));
#7279=DIRECTION('center_axis',(0.,-1.,0.));
#7280=DIRECTION('ref_axis',(1.,0.,0.));
#7281=DIRECTION('center_axis',(0.,1.,0.));
#7282=DIRECTION('ref_axis',(-1.,0.,3.21624529935327E-16));
#7283=DIRECTION('center_axis',(0.,-1.,0.));
#7284=DIRECTION('ref_axis',(1.,0.,0.));
#7285=DIRECTION('',(0.,-1.,0.));
#7286=DIRECTION('center_axis',(-0.866025403784439,0.,-0.5));
#7287=DIRECTION('ref_axis',(-0.5,0.,0.866025403784439));
#7288=DIRECTION('',(-0.5,0.,0.866025403784439));
#7289=DIRECTION('',(0.,1.,0.));
#7290=DIRECTION('center_axis',(0.866025403784439,0.,0.5));
#7291=DIRECTION('ref_axis',(0.5,0.,-0.866025403784439));
#7292=DIRECTION('',(0.,1.,0.));
#7293=DIRECTION('',(0.,-1.,0.));
#7294=DIRECTION('',(0.5,0.,-0.866025403784439));
#7295=DIRECTION('center_axis',(0.,1.,0.));
#7296=DIRECTION('ref_axis',(1.,0.,0.));
#7297=DIRECTION('center_axis',(0.,-1.,0.));
#7298=DIRECTION('ref_axis',(1.,0.,0.));
#7299=DIRECTION('',(0.,-1.,0.));
#7300=DIRECTION('center_axis',(0.,0.,1.));
#7301=DIRECTION('ref_axis',(1.,0.,0.));
#7302=DIRECTION('',(0.,1.,0.));
#7303=DIRECTION('',(1.,0.,0.));
#7304=DIRECTION('center_axis',(0.,0.,-1.));
#7305=DIRECTION('ref_axis',(-1.,0.,0.));
#7306=DIRECTION('',(0.,-1.,0.));
#7307=DIRECTION('',(-1.,0.,0.));
#7308=DIRECTION('',(0.,1.,0.));
#7309=DIRECTION('center_axis',(0.,1.,0.));
#7310=DIRECTION('ref_axis',(1.,0.,0.));
#7311=DIRECTION('center_axis',(0.,1.,0.));
#7312=DIRECTION('ref_axis',(1.,0.,0.));
#7313=DIRECTION('center_axis',(0.,-1.,0.));
#7314=DIRECTION('ref_axis',(1.,0.,0.));
#7315=DIRECTION('center_axis',(0.,1.,0.));
#7316=DIRECTION('ref_axis',(1.,0.,0.));
#7317=DIRECTION('center_axis',(0.,1.,0.));
#7318=DIRECTION('ref_axis',(1.,0.,0.));
#7319=DIRECTION('center_axis',(0.,1.,0.));
#7320=DIRECTION('ref_axis',(1.,0.,0.));
#7321=DIRECTION('center_axis',(0.,1.,0.));
#7322=DIRECTION('ref_axis',(1.,0.,0.));
#7323=DIRECTION('center_axis',(0.,1.,0.));
#7324=DIRECTION('ref_axis',(1.,0.,0.));
#7325=DIRECTION('',(0.,-1.,0.));
#7326=DIRECTION('center_axis',(0.,1.,0.));
#7327=DIRECTION('ref_axis',(1.,0.,0.));
#7328=DIRECTION('',(0.,-1.,0.));
#7329=DIRECTION('center_axis',(0.,1.,0.));
#7330=DIRECTION('ref_axis',(1.,0.,0.));
#7331=DIRECTION('center_axis',(0.,1.,0.));
#7332=DIRECTION('ref_axis',(1.,0.,0.));
#9148=CARTESIAN_POINT('',(0.,0.,0.));
#9149=CARTESIAN_POINT('Origin',(5.3,-3.1,10.));
#9150=CARTESIAN_POINT('',(5.135,-3.,10.));
#9151=CARTESIAN_POINT('Origin',(5.3,-3.,10.));
#9152=CARTESIAN_POINT('',(5.135,-2.2,10.));
#9153=CARTESIAN_POINT('',(5.135,-3.1,10.));
#9154=CARTESIAN_POINT('Origin',(5.3,-2.2,10.));
#9155=CARTESIAN_POINT('Origin',(7.7,-3.1,10.));
#9156=CARTESIAN_POINT('',(7.535,-3.,10.));
#9157=CARTESIAN_POINT('Origin',(7.7,-3.,10.));
#9158=CARTESIAN_POINT('',(7.535,-2.2,10.));
#9159=CARTESIAN_POINT('',(7.535,-3.1,10.));
#9160=CARTESIAN_POINT('Origin',(7.7,-2.2,10.));
#9161=CARTESIAN_POINT('Origin',(0.,-2.,10.59));
#9162=CARTESIAN_POINT('',(0.109087121146348,-2.17944358444927,10.59));
#9163=CARTESIAN_POINT('',(0.109087121146348,-1.82055641555073,10.59));
#9164=CARTESIAN_POINT('',(0.109087121146348,-3.5,10.59));
#9165=CARTESIAN_POINT('Origin',(0.,-2.,10.59));
#9166=CARTESIAN_POINT('Origin',(0.,-2.,10.59));
#9167=CARTESIAN_POINT('',(-0.109087121146348,-2.17944358444927,10.59));
#9168=CARTESIAN_POINT('Ctrl Pts',(-0.109087121146349,-2.17944358444927,
10.59));
#9169=CARTESIAN_POINT('Ctrl Pts',(-0.100058962329428,-2.18493197155217,
10.5916692472112));
#9170=CARTESIAN_POINT('Ctrl Pts',(-0.0905297208284635,-2.18978489888129,
10.5932143633855));
#9171=CARTESIAN_POINT('Ctrl Pts',(-0.0548356965671432,-2.20463697075952,
10.598057680137));
#9172=CARTESIAN_POINT('Ctrl Pts',(-0.0266060994851221,-2.21,10.6));
#9173=CARTESIAN_POINT('Ctrl Pts',(0.026606099485122,-2.21,10.6));
#9174=CARTESIAN_POINT('Ctrl Pts',(0.0548356965671431,-2.20463697075952,
10.598057680137));
#9175=CARTESIAN_POINT('Ctrl Pts',(0.0905297208284635,-2.18978489888129,
10.5932143633855));
#9176=CARTESIAN_POINT('Ctrl Pts',(0.100058962329428,-2.18493197155217,10.5916692472112));
#9177=CARTESIAN_POINT('Ctrl Pts',(0.109087121146348,-2.17944358444927,10.59));
#9178=CARTESIAN_POINT('',(-0.21,-2.,10.59));
#9179=CARTESIAN_POINT('Origin',(0.,-2.,10.59));
#9180=CARTESIAN_POINT('',(-0.21,-2.,11.4852272553384));
#9181=CARTESIAN_POINT('',(-0.21,-2.,10.59));
#9182=CARTESIAN_POINT('',(0.21,-2.,11.4852272553384));
#9183=CARTESIAN_POINT('Ctrl Pts',(0.21,-2.,11.4852272553384));
#9184=CARTESIAN_POINT('Ctrl Pts',(0.21,-2.02640552692445,11.4852272553384));
#9185=CARTESIAN_POINT('Ctrl Pts',(0.204715737269596,-2.05454707409071,11.4860041595441));
#9186=CARTESIAN_POINT('Ctrl Pts',(0.183273763036332,-2.10627626890513,11.4888007328232));
#9187=CARTESIAN_POINT('Ctrl Pts',(0.167117923970394,-2.12986692412796,11.4907789715758));
#9188=CARTESIAN_POINT('Ctrl Pts',(0.129867169887369,-2.16711767821098,11.4944848114133));
#9189=CARTESIAN_POINT('Ctrl Pts',(0.106276408305765,-2.18327371000135,11.4964545565713));
#9190=CARTESIAN_POINT('Ctrl Pts',(0.0545468514059001,-2.20471582482622,
11.4992316551565));
#9191=CARTESIAN_POINT('Ctrl Pts',(0.0264051785092814,-2.21,11.5));
#9192=CARTESIAN_POINT('Ctrl Pts',(-0.0264051785092814,-2.21,11.5));
#9193=CARTESIAN_POINT('Ctrl Pts',(-0.0545468514059001,-2.20471582482622,
11.4992316551565));
#9194=CARTESIAN_POINT('Ctrl Pts',(-0.106276408305765,-2.18327371000135,
11.4964545565713));
#9195=CARTESIAN_POINT('Ctrl Pts',(-0.129867169887369,-2.16711767821098,
11.4944848114133));
#9196=CARTESIAN_POINT('Ctrl Pts',(-0.167117923970394,-2.12986692412796,
11.4907789715758));
#9197=CARTESIAN_POINT('Ctrl Pts',(-0.183273763036332,-2.10627626890513,
11.4888007328232));
#9198=CARTESIAN_POINT('Ctrl Pts',(-0.204715737269596,-2.05454707409071,
11.4860041595441));
#9199=CARTESIAN_POINT('Ctrl Pts',(-0.21,-2.02640552692445,11.4852272553384));
#9200=CARTESIAN_POINT('Ctrl Pts',(-0.21,-2.,11.4852272553384));
#9201=CARTESIAN_POINT('Ctrl Pts',(-0.21,-2.,11.4852272553384));
#9202=CARTESIAN_POINT('Ctrl Pts',(-0.21,-1.97359447307555,11.4852272553384));
#9203=CARTESIAN_POINT('Ctrl Pts',(-0.204715737269596,-1.94545292590929,
11.4860041595441));
#9204=CARTESIAN_POINT('Ctrl Pts',(-0.183273763036331,-1.89372373109487,
11.4888007328232));
#9205=CARTESIAN_POINT('Ctrl Pts',(-0.167117923970394,-1.87013307587204,
11.4907789715758));
#9206=CARTESIAN_POINT('Ctrl Pts',(-0.129867169887369,-1.83288232178902,
11.4944848114133));
#9207=CARTESIAN_POINT('Ctrl Pts',(-0.106276408305765,-1.81672628999865,
11.4964545565713));
#9208=CARTESIAN_POINT('Ctrl Pts',(-0.0545468514059002,-1.79528417517378,
11.4992316551565));
#9209=CARTESIAN_POINT('Ctrl Pts',(-0.0264051785092814,-1.79,11.5));
#9210=CARTESIAN_POINT('Ctrl Pts',(0.0264051785092814,-1.79,11.5));
#9211=CARTESIAN_POINT('Ctrl Pts',(0.0545468514059001,-1.79528417517378,
11.4992316551565));
#9212=CARTESIAN_POINT('Ctrl Pts',(0.106276408305765,-1.81672628999865,11.4964545565713));
#9213=CARTESIAN_POINT('Ctrl Pts',(0.129867169887369,-1.83288232178902,11.4944848114133));
#9214=CARTESIAN_POINT('Ctrl Pts',(0.167117923970394,-1.87013307587204,11.4907789715758));
#9215=CARTESIAN_POINT('Ctrl Pts',(0.183273763036331,-1.89372373109487,11.4888007328232));
#9216=CARTESIAN_POINT('Ctrl Pts',(0.204715737269596,-1.94545292590929,11.4860041595441));
#9217=CARTESIAN_POINT('Ctrl Pts',(0.21,-1.97359447307555,11.4852272553384));
#9218=CARTESIAN_POINT('Ctrl Pts',(0.21,-2.,11.4852272553384));
#9219=CARTESIAN_POINT('',(-0.109087121146348,-1.82055641555073,10.59));
#9220=CARTESIAN_POINT('Origin',(0.,-2.,10.59));
#9221=CARTESIAN_POINT('Ctrl Pts',(0.109087121146348,-1.82055641555073,10.59));
#9222=CARTESIAN_POINT('Ctrl Pts',(0.100058962329427,-1.81506802844783,10.5916692472112));
#9223=CARTESIAN_POINT('Ctrl Pts',(0.0905297208284631,-1.81021510111871,
10.5932143633855));
#9224=CARTESIAN_POINT('Ctrl Pts',(0.054835696567143,-1.79536302924048,10.598057680137));
#9225=CARTESIAN_POINT('Ctrl Pts',(0.026606099485122,-1.79,10.6));
#9226=CARTESIAN_POINT('Ctrl Pts',(-0.026606099485122,-1.79,10.6));
#9227=CARTESIAN_POINT('Ctrl Pts',(-0.0548356965671429,-1.79536302924048,
10.598057680137));
#9228=CARTESIAN_POINT('Ctrl Pts',(-0.0905297208284631,-1.81021510111871,
10.5932143633855));
#9229=CARTESIAN_POINT('Ctrl Pts',(-0.100058962329428,-1.81506802844783,
10.5916692472112));
#9230=CARTESIAN_POINT('Ctrl Pts',(-0.109087121146348,-1.82055641555073,
10.59));
#9231=CARTESIAN_POINT('Origin',(0.,-2.,10.59));
#9232=CARTESIAN_POINT('',(-0.109087121146348,-3.5,10.59));
#9233=CARTESIAN_POINT('Origin',(-0.2,-3.6,9.22));
#9234=CARTESIAN_POINT('',(-0.2,-3.5,9.22));
#9235=CARTESIAN_POINT('',(-0.2,-3.5,9.43431457505076));
#9236=CARTESIAN_POINT('',(-0.2,-3.5,9.61));
#9237=CARTESIAN_POINT('',(-0.2,-1.5,9.22));
#9238=CARTESIAN_POINT('',(-0.2,-3.6,9.22));
#9239=CARTESIAN_POINT('',(-0.2,-1.5,9.43431457505076));
#9240=CARTESIAN_POINT('',(-0.2,-1.5,9.61));
#9241=CARTESIAN_POINT('',(-0.2,-3.5,9.43431457505076));
#9242=CARTESIAN_POINT('Origin',(0.2,-3.6,9.22));
#9243=CARTESIAN_POINT('',(0.2,-3.5,9.22));
#9244=CARTESIAN_POINT('',(0.1,-3.5,9.22));
#9245=CARTESIAN_POINT('',(0.2,-1.5,9.22));
#9246=CARTESIAN_POINT('',(0.2,-3.6,9.22));
#9247=CARTESIAN_POINT('',(0.1,-1.5,9.22));
#9248=CARTESIAN_POINT('Origin',(0.2,-3.6,10.));
#9249=CARTESIAN_POINT('',(0.2,-3.5,9.43431457505076));
#9250=CARTESIAN_POINT('',(0.2,-3.5,10.));
#9251=CARTESIAN_POINT('',(0.2,-1.5,9.43431457505076));
#9252=CARTESIAN_POINT('',(0.2,-3.5,9.43431457505076));
#9253=CARTESIAN_POINT('',(0.2,-1.5,10.));
#9254=CARTESIAN_POINT('Origin',(0.,-1.5,10.));
#9255=CARTESIAN_POINT('',(-1.5,-1.5,10.));
#9256=CARTESIAN_POINT('Origin',(0.,-1.5,10.));
#9257=CARTESIAN_POINT('Origin',(0.,-1.5,10.));
#9258=CARTESIAN_POINT('Origin',(0.,-3.5,10.));
#9259=CARTESIAN_POINT('Origin',(0.,-3.5,10.));
#9260=CARTESIAN_POINT('Origin',(-0.266987298107781,-3.,8.53756443470179));
#9261=CARTESIAN_POINT('',(-3.18335633348014,-2.2,3.48626509181623));
#9262=CARTESIAN_POINT('',(-3.18335633348014,-3.,3.48626509181623));
#9263=CARTESIAN_POINT('',(-3.18335633348014,-3.,3.48626509181623));
#9264=CARTESIAN_POINT('',(-0.27409407929433,-2.2,8.52525512860841));
#9265=CARTESIAN_POINT('',(-3.26698729810778,-2.2,3.34141201199516));
#9266=CARTESIAN_POINT('',(-0.27409407929433,-3.,8.52525512860841));
#9267=CARTESIAN_POINT('',(-0.274094079294329,-3.5,8.52525512860841));
#9268=CARTESIAN_POINT('',(-3.26698729810778,-3.,3.34141201199516));
#9269=CARTESIAN_POINT('Origin',(-4.13301270189222,-3.,3.84141201199516));
#9270=CARTESIAN_POINT('',(-4.04938173726458,-3.,3.98626509181623));
#9271=CARTESIAN_POINT('',(-4.04938173726458,-2.2,3.98626509181623));
#9272=CARTESIAN_POINT('',(-4.04938173726458,-3.,3.98626509181623));
#9273=CARTESIAN_POINT('',(-1.14011948307877,-3.,9.02525512860841));
#9274=CARTESIAN_POINT('',(-1.13301270189222,-3.,9.03756443470179));
#9275=CARTESIAN_POINT('',(-1.14011948307877,-2.2,9.02525512860841));
#9276=CARTESIAN_POINT('',(-1.14011948307877,-3.5,9.02525512860841));
#9277=CARTESIAN_POINT('',(-1.13301270189222,-2.2,9.03756443470179));
#9278=CARTESIAN_POINT('Origin',(0.,-3.,10.));
#9279=CARTESIAN_POINT('',(-8.,-3.,10.));
#9280=CARTESIAN_POINT('Origin',(0.,-3.,10.));
#9281=CARTESIAN_POINT('',(-4.04938173726458,-3.,16.0137349081838));
#9282=CARTESIAN_POINT('Origin',(0.,-3.,10.));
#9283=CARTESIAN_POINT('',(-1.14011948307877,-3.,10.9747448713916));
#9284=CARTESIAN_POINT('',(-4.13301270189222,-3.,16.1585879880048));
#9285=CARTESIAN_POINT('',(-0.274094079294328,-3.,11.4747448713916));
#9286=CARTESIAN_POINT('Origin',(0.,-3.,10.));
#9287=CARTESIAN_POINT('',(-3.18335633348014,-3.,16.5137349081838));
#9288=CARTESIAN_POINT('',(-0.26698729810778,-3.,11.4624355652982));
#9289=CARTESIAN_POINT('',(7.23273807074472,-3.,10.5));
#9290=CARTESIAN_POINT('Origin',(0.,-3.,10.));
#9291=CARTESIAN_POINT('',(1.4142135623731,-3.,10.5));
#9292=CARTESIAN_POINT('',(7.4,-3.,10.5));
#9293=CARTESIAN_POINT('',(1.4142135623731,-3.,9.5));
#9294=CARTESIAN_POINT('Origin',(0.,-3.,10.));
#9295=CARTESIAN_POINT('',(7.23273807074472,-3.,9.5));
#9296=CARTESIAN_POINT('',(1.4,-3.,9.5));
#9297=CARTESIAN_POINT('Origin',(0.,-3.,10.));
#9298=CARTESIAN_POINT('Origin',(0.,-3.,10.));
#9299=CARTESIAN_POINT('Origin',(0.,-3.,10.));
#9300=CARTESIAN_POINT('',(-4.04938173726458,-2.2,16.0137349081838));
#9301=CARTESIAN_POINT('Origin',(0.,-2.2,10.));
#9302=CARTESIAN_POINT('',(-4.04938173726458,-3.,16.0137349081838));
#9303=CARTESIAN_POINT('Origin',(-1.13301270189222,-3.,10.9624355652982));
#9304=CARTESIAN_POINT('',(-1.14011948307877,-2.2,10.9747448713916));
#9305=CARTESIAN_POINT('',(-4.13301270189222,-2.2,16.1585879880048));
#9306=CARTESIAN_POINT('',(-1.14011948307877,-3.5,10.9747448713916));
#9307=CARTESIAN_POINT('Origin',(-3.26698729810778,-3.,16.6585879880048));
#9308=CARTESIAN_POINT('',(-3.18335633348014,-2.2,16.5137349081838));
#9309=CARTESIAN_POINT('',(-3.18335633348014,-3.,16.5137349081838));
#9310=CARTESIAN_POINT('',(-0.274094079294328,-2.2,11.4747448713916));
#9311=CARTESIAN_POINT('',(-0.274094079294328,-3.5,11.4747448713916));
#9312=CARTESIAN_POINT('',(-0.26698729810778,-2.2,11.4624355652982));
#9313=CARTESIAN_POINT('Origin',(0.,-3.,10.));
#9314=CARTESIAN_POINT('',(7.23273807074472,-2.2,10.5));
#9315=CARTESIAN_POINT('Origin',(0.,-2.2,10.));
#9316=CARTESIAN_POINT('',(7.23273807074472,-3.,10.5));
#9317=CARTESIAN_POINT('Origin',(1.4,-3.,10.5));
#9318=CARTESIAN_POINT('',(1.4142135623731,-2.2,10.5));
#9319=CARTESIAN_POINT('',(1.4142135623731,-3.5,10.5));
#9320=CARTESIAN_POINT('',(7.4,-2.2,10.5));
#9321=CARTESIAN_POINT('Origin',(7.4,-3.,9.5));
#9322=CARTESIAN_POINT('',(1.4142135623731,-2.2,9.5));
#9323=CARTESIAN_POINT('',(1.4142135623731,-3.5,9.5));
#9324=CARTESIAN_POINT('',(7.23273807074472,-2.2,9.5));
#9325=CARTESIAN_POINT('',(1.4,-2.2,9.5));
#9326=CARTESIAN_POINT('',(7.23273807074472,-3.,9.5));
#9327=CARTESIAN_POINT('Origin',(0.,-2.2,10.));
#9328=CARTESIAN_POINT('',(-8.,-2.2,10.));
#9329=CARTESIAN_POINT('Origin',(0.,-2.2,10.));
#9330=CARTESIAN_POINT('Origin',(0.,-2.2,10.));
#9331=CARTESIAN_POINT('Origin',(0.,-2.2,10.));
#9332=CARTESIAN_POINT('Origin',(0.,-2.2,10.));
#9333=CARTESIAN_POINT('Origin',(0.,-2.2,10.));
#9334=CARTESIAN_POINT('Origin',(0.,-3.,10.));
#9335=CARTESIAN_POINT('Origin',(0.,-3.,10.));
#9336=CARTESIAN_POINT('',(-8.,-3.,10.));
#9337=CARTESIAN_POINT('Origin',(0.,-3.5,10.));
#9338=CARTESIAN_POINT('',(-1.5,-3.5,10.));
#9339=CARTESIAN_POINT('',(-1.5,-3.5,10.));
#9340=CARTESIAN_POINT('Origin',(0.,-3.5,10.));
#9341=CARTESIAN_POINT('Origin',(0.,-3.5,10.));
#10452=UNCERTAINTY_MEASURE_WITH_UNIT(LENGTH_MEASURE(0.001),#10511,
'DISTANCE_ACCURACY_VALUE',
'Maximum model space distance between geometric entities at asserted c
onnectivities');
#10471=UNCERTAINTY_MEASURE_WITH_UNIT(LENGTH_MEASURE(0.001),#10511,
'DISTANCE_ACCURACY_VALUE',
'Maximum model space distance between geometric entities at asserted c
onnectivities');
#10491=(
GEOMETRIC_REPRESENTATION_CONTEXT(3)
GLOBAL_UNCERTAINTY_ASSIGNED_CONTEXT((#10452))
GLOBAL_UNIT_ASSIGNED_CONTEXT((#10511,#10513,#10514))
REPRESENTATION_CONTEXT('','3D')
);
#10510=(
GEOMETRIC_REPRESENTATION_CONTEXT(3)
GLOBAL_UNCERTAINTY_ASSIGNED_CONTEXT((#10471))
GLOBAL_UNIT_ASSIGNED_CONTEXT((#10511,#10513,#10514))
REPRESENTATION_CONTEXT('','3D')
);
#10511=(
LENGTH_UNIT()
NAMED_UNIT(*)
SI_UNIT(.CENTI.,.METRE.)
);
#10513=(
NAMED_UNIT(*)
PLANE_ANGLE_UNIT()
SI_UNIT($,.RADIAN.)
);
#10514=(
NAMED_UNIT(*)
SI_UNIT($,.STERADIAN.)
SOLID_ANGLE_UNIT()
);
#10534=SHAPE_DEFINITION_REPRESENTATION(#10577,#10664);
#10577=PRODUCT_DEFINITION_SHAPE('',$,#10703);
#10664=SHAPE_REPRESENTATION('',(#6012),#10491);
#10683=PRODUCT_DEFINITION_CONTEXT('part definition',#10799,'design');
#10703=PRODUCT_DEFINITION('Hand wheel','Hand wheel',#10741,#10683);
#10741=PRODUCT_DEFINITION_FORMATION('',$,#10820);
#10799=APPLICATION_CONTEXT(
'Core Data for Automotive Mechanical Design Process');
#10800=PRODUCT_CONTEXT('part definition',#10799,'mechanical');
#10820=PRODUCT('Hand wheel','Hand wheel','Hand wheel',(#10800));
#10895=COLOUR_RGB('Sky Blue',0.24,0.69,0.87);
#10896=FILL_AREA_STYLE_COLOUR('',#10895);
#10897=FILL_AREA_STYLE('',(#10896));
#10898=SURFACE_STYLE_FILL_AREA(#10897);
#10899=SURFACE_SIDE_STYLE('',(#10898));
#10900=SURFACE_STYLE_USAGE(.BOTH.,#10899);
#10901=PRESENTATION_STYLE_ASSIGNMENT((#10900));
ENDSEC;
END-ISO-10303-21;
